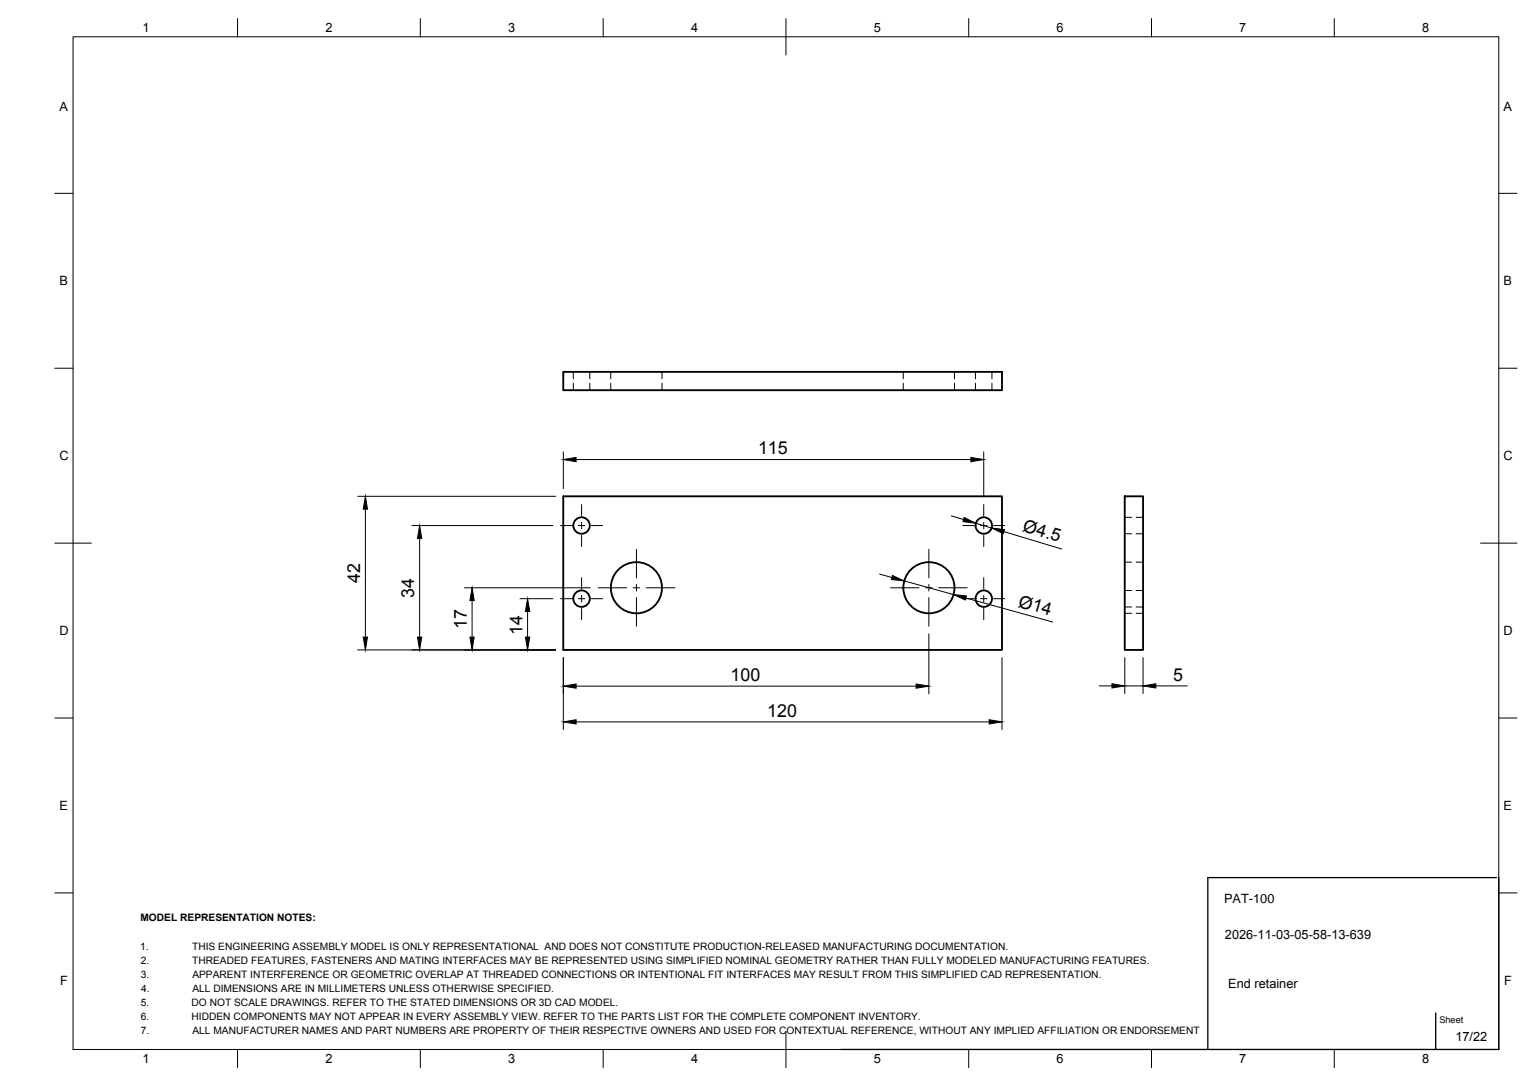
ISO-10303-21;
HEADER;
/* Generated by software containing ST-Developer
 * from STEP Tools, Inc. (www.steptools.com) 
 */

FILE_DESCRIPTION(
/* description */ (''),
/* implementation_level */ '2;1');

FILE_NAME(
/* name */ 'End retainer.step',
/* time_stamp */ '2026-10-29T16:43:51-07:00',
/* author */ (''),
/* organization */ (''),
/* preprocessor_version */ 'ST-DEVELOPER v20.2',
/* originating_system */ 'Autodesk Translation Framework v15.17.0.0',
/* authorisation */ '');

FILE_SCHEMA (('AUTOMOTIVE_DESIGN { 1 0 10303 214 3 1 1 }'));
ENDSEC;

DATA;
#10=MECHANICAL_DESIGN_GEOMETRIC_PRESENTATION_REPRESENTATION('',(#382),#10292);
#336=SHAPE_REPRESENTATION_RELATIONSHIP('SRR','None',#10434,#359);
#359=ADVANCED_BREP_SHAPE_REPRESENTATION('',(#403),#10286);
#382=STYLED_ITEM('',(#10614),#403);
#403=MANIFOLD_SOLID_BREP('Body1',#5026);
#512=FACE_BOUND('',#1329,.T.);
#513=FACE_BOUND('',#1330,.T.);
#514=FACE_BOUND('',#1331,.T.);
#515=FACE_BOUND('',#1332,.T.);
#516=FACE_BOUND('',#1333,.T.);
#517=FACE_BOUND('',#1334,.T.);
#518=FACE_BOUND('',#1337,.T.);
#519=FACE_BOUND('',#1338,.T.);
#520=FACE_BOUND('',#1339,.T.);
#521=FACE_BOUND('',#1340,.T.);
#522=FACE_BOUND('',#1341,.T.);
#523=FACE_BOUND('',#1342,.T.);
#667=PLANE('',#5702);
#668=PLANE('',#5703);
#669=PLANE('',#5704);
#670=PLANE('',#5705);
#671=PLANE('',#5706);
#672=PLANE('',#5707);
#927=FACE_OUTER_BOUND('',#1321,.T.);
#928=FACE_OUTER_BOUND('',#1322,.T.);
#929=FACE_OUTER_BOUND('',#1323,.T.);
#930=FACE_OUTER_BOUND('',#1324,.T.);
#931=FACE_OUTER_BOUND('',#1325,.T.);
#932=FACE_OUTER_BOUND('',#1326,.T.);
#933=FACE_OUTER_BOUND('',#1327,.T.);
#934=FACE_OUTER_BOUND('',#1328,.T.);
#935=FACE_OUTER_BOUND('',#1335,.T.);
#936=FACE_OUTER_BOUND('',#1336,.T.);
#937=FACE_OUTER_BOUND('',#1343,.T.);
#938=FACE_OUTER_BOUND('',#1344,.T.);
#1321=EDGE_LOOP('',(#4361,#4362,#4363,#4364));
#1322=EDGE_LOOP('',(#4365,#4366,#4367,#4368));
#1323=EDGE_LOOP('',(#4369,#4370,#4371,#4372));
#1324=EDGE_LOOP('',(#4373,#4374,#4375,#4376));
#1325=EDGE_LOOP('',(#4377,#4378,#4379,#4380));
#1326=EDGE_LOOP('',(#4381,#4382,#4383,#4384));
#1327=EDGE_LOOP('',(#4385,#4386,#4387,#4388));
#1328=EDGE_LOOP('',(#4389,#4390,#4391,#4392));
#1329=EDGE_LOOP('',(#4393));
#1330=EDGE_LOOP('',(#4394));
#1331=EDGE_LOOP('',(#4395));
#1332=EDGE_LOOP('',(#4396));
#1333=EDGE_LOOP('',(#4397));
#1334=EDGE_LOOP('',(#4398));
#1335=EDGE_LOOP('',(#4399,#4400,#4401,#4402));
#1336=EDGE_LOOP('',(#4403,#4404,#4405,#4406));
#1337=EDGE_LOOP('',(#4407));
#1338=EDGE_LOOP('',(#4408));
#1339=EDGE_LOOP('',(#4409));
#1340=EDGE_LOOP('',(#4410));
#1341=EDGE_LOOP('',(#4411));
#1342=EDGE_LOOP('',(#4412));
#1343=EDGE_LOOP('',(#4413,#4414,#4415,#4416));
#1344=EDGE_LOOP('',(#4417,#4418,#4419,#4420));
#1709=LINE('',#9879,#2101);
#1710=LINE('',#9885,#2102);
#1711=LINE('',#9891,#2103);
#1712=LINE('',#9897,#2104);
#1713=LINE('',#9903,#2105);
#1714=LINE('',#9909,#2106);
#1715=LINE('',#9914,#2107);
#1716=LINE('',#9916,#2108);
#1717=LINE('',#9918,#2109);
#1718=LINE('',#9919,#2110);
#1719=LINE('',#9922,#2111);
#1720=LINE('',#9924,#2112);
#1721=LINE('',#9925,#2113);
#1722=LINE('',#9928,#2114);
#1723=LINE('',#9930,#2115);
#1724=LINE('',#9931,#2116);
#1725=LINE('',#9933,#2117);
#1726=LINE('',#9934,#2118);
#2101=VECTOR('',#6956,0.225);
#2102=VECTOR('',#6963,0.225);
#2103=VECTOR('',#6970,0.225);
#2104=VECTOR('',#6977,0.225);
#2105=VECTOR('',#6984,0.7);
#2106=VECTOR('',#6991,0.7);
#2107=VECTOR('',#6996,1.);
#2108=VECTOR('',#6997,1.);
#2109=VECTOR('',#6998,1.);
#2110=VECTOR('',#6999,1.);
#2111=VECTOR('',#7002,1.);
#2112=VECTOR('',#7003,1.);
#2113=VECTOR('',#7004,1.);
#2114=VECTOR('',#7007,1.);
#2115=VECTOR('',#7008,1.);
#2116=VECTOR('',#7009,1.);
#2117=VECTOR('',#7012,1.);
#2118=VECTOR('',#7013,1.);
#2350=CIRCLE('',#5685,0.225);
#2351=CIRCLE('',#5686,0.225);
#2352=CIRCLE('',#5688,0.225);
#2353=CIRCLE('',#5689,0.225);
#2354=CIRCLE('',#5691,0.225);
#2355=CIRCLE('',#5692,0.225);
#2356=CIRCLE('',#5694,0.225);
#2357=CIRCLE('',#5695,0.225);
#2358=CIRCLE('',#5697,0.7);
#2359=CIRCLE('',#5698,0.7);
#2360=CIRCLE('',#5700,0.7);
#2361=CIRCLE('',#5701,0.7);
#2707=VERTEX_POINT('',#9876);
#2708=VERTEX_POINT('',#9878);
#2709=VERTEX_POINT('',#9882);
#2710=VERTEX_POINT('',#9884);
#2711=VERTEX_POINT('',#9888);
#2712=VERTEX_POINT('',#9890);
#2713=VERTEX_POINT('',#9894);
#2714=VERTEX_POINT('',#9896);
#2715=VERTEX_POINT('',#9900);
#2716=VERTEX_POINT('',#9902);
#2717=VERTEX_POINT('',#9906);
#2718=VERTEX_POINT('',#9908);
#2719=VERTEX_POINT('',#9912);
#2720=VERTEX_POINT('',#9913);
#2721=VERTEX_POINT('',#9915);
#2722=VERTEX_POINT('',#9917);
#2723=VERTEX_POINT('',#9921);
#2724=VERTEX_POINT('',#9923);
#2725=VERTEX_POINT('',#9927);
#2726=VERTEX_POINT('',#9929);
#3271=EDGE_CURVE('',#2707,#2707,#2350,.T.);
#3272=EDGE_CURVE('',#2707,#2708,#1709,.T.);
#3273=EDGE_CURVE('',#2708,#2708,#2351,.T.);
#3274=EDGE_CURVE('',#2709,#2709,#2352,.T.);
#3275=EDGE_CURVE('',#2709,#2710,#1710,.T.);
#3276=EDGE_CURVE('',#2710,#2710,#2353,.T.);
#3277=EDGE_CURVE('',#2711,#2711,#2354,.T.);
#3278=EDGE_CURVE('',#2711,#2712,#1711,.T.);
#3279=EDGE_CURVE('',#2712,#2712,#2355,.T.);
#3280=EDGE_CURVE('',#2713,#2713,#2356,.T.);
#3281=EDGE_CURVE('',#2713,#2714,#1712,.T.);
#3282=EDGE_CURVE('',#2714,#2714,#2357,.T.);
#3283=EDGE_CURVE('',#2715,#2715,#2358,.T.);
#3284=EDGE_CURVE('',#2715,#2716,#1713,.T.);
#3285=EDGE_CURVE('',#2716,#2716,#2359,.T.);
#3286=EDGE_CURVE('',#2717,#2717,#2360,.T.);
#3287=EDGE_CURVE('',#2717,#2718,#1714,.T.);
#3288=EDGE_CURVE('',#2718,#2718,#2361,.T.);
#3289=EDGE_CURVE('',#2719,#2720,#1715,.T.);
#3290=EDGE_CURVE('',#2720,#2721,#1716,.T.);
#3291=EDGE_CURVE('',#2722,#2721,#1717,.T.);
#3292=EDGE_CURVE('',#2719,#2722,#1718,.T.);
#3293=EDGE_CURVE('',#2723,#2719,#1719,.T.);
#3294=EDGE_CURVE('',#2724,#2722,#1720,.T.);
#3295=EDGE_CURVE('',#2723,#2724,#1721,.T.);
#3296=EDGE_CURVE('',#2725,#2723,#1722,.T.);
#3297=EDGE_CURVE('',#2726,#2724,#1723,.T.);
#3298=EDGE_CURVE('',#2725,#2726,#1724,.T.);
#3299=EDGE_CURVE('',#2720,#2725,#1725,.T.);
#3300=EDGE_CURVE('',#2721,#2726,#1726,.T.);
#4361=ORIENTED_EDGE('',*,*,#3271,.F.);
#4362=ORIENTED_EDGE('',*,*,#3272,.T.);
#4363=ORIENTED_EDGE('',*,*,#3273,.F.);
#4364=ORIENTED_EDGE('',*,*,#3272,.F.);
#4365=ORIENTED_EDGE('',*,*,#3274,.F.);
#4366=ORIENTED_EDGE('',*,*,#3275,.T.);
#4367=ORIENTED_EDGE('',*,*,#3276,.F.);
#4368=ORIENTED_EDGE('',*,*,#3275,.F.);
#4369=ORIENTED_EDGE('',*,*,#3277,.F.);
#4370=ORIENTED_EDGE('',*,*,#3278,.T.);
#4371=ORIENTED_EDGE('',*,*,#3279,.F.);
#4372=ORIENTED_EDGE('',*,*,#3278,.F.);
#4373=ORIENTED_EDGE('',*,*,#3280,.F.);
#4374=ORIENTED_EDGE('',*,*,#3281,.T.);
#4375=ORIENTED_EDGE('',*,*,#3282,.F.);
#4376=ORIENTED_EDGE('',*,*,#3281,.F.);
#4377=ORIENTED_EDGE('',*,*,#3283,.F.);
#4378=ORIENTED_EDGE('',*,*,#3284,.T.);
#4379=ORIENTED_EDGE('',*,*,#3285,.F.);
#4380=ORIENTED_EDGE('',*,*,#3284,.F.);
#4381=ORIENTED_EDGE('',*,*,#3286,.F.);
#4382=ORIENTED_EDGE('',*,*,#3287,.T.);
#4383=ORIENTED_EDGE('',*,*,#3288,.F.);
#4384=ORIENTED_EDGE('',*,*,#3287,.F.);
#4385=ORIENTED_EDGE('',*,*,#3289,.T.);
#4386=ORIENTED_EDGE('',*,*,#3290,.T.);
#4387=ORIENTED_EDGE('',*,*,#3291,.F.);
#4388=ORIENTED_EDGE('',*,*,#3292,.F.);
#4389=ORIENTED_EDGE('',*,*,#3293,.T.);
#4390=ORIENTED_EDGE('',*,*,#3292,.T.);
#4391=ORIENTED_EDGE('',*,*,#3294,.F.);
#4392=ORIENTED_EDGE('',*,*,#3295,.F.);
#4393=ORIENTED_EDGE('',*,*,#3288,.T.);
#4394=ORIENTED_EDGE('',*,*,#3285,.T.);
#4395=ORIENTED_EDGE('',*,*,#3282,.T.);
#4396=ORIENTED_EDGE('',*,*,#3279,.T.);
#4397=ORIENTED_EDGE('',*,*,#3276,.T.);
#4398=ORIENTED_EDGE('',*,*,#3273,.T.);
#4399=ORIENTED_EDGE('',*,*,#3296,.T.);
#4400=ORIENTED_EDGE('',*,*,#3295,.T.);
#4401=ORIENTED_EDGE('',*,*,#3297,.F.);
#4402=ORIENTED_EDGE('',*,*,#3298,.F.);
#4403=ORIENTED_EDGE('',*,*,#3299,.T.);
#4404=ORIENTED_EDGE('',*,*,#3298,.T.);
#4405=ORIENTED_EDGE('',*,*,#3300,.F.);
#4406=ORIENTED_EDGE('',*,*,#3290,.F.);
#4407=ORIENTED_EDGE('',*,*,#3286,.T.);
#4408=ORIENTED_EDGE('',*,*,#3283,.T.);
#4409=ORIENTED_EDGE('',*,*,#3280,.T.);
#4410=ORIENTED_EDGE('',*,*,#3277,.T.);
#4411=ORIENTED_EDGE('',*,*,#3274,.T.);
#4412=ORIENTED_EDGE('',*,*,#3271,.T.);
#4413=ORIENTED_EDGE('',*,*,#3300,.T.);
#4414=ORIENTED_EDGE('',*,*,#3297,.T.);
#4415=ORIENTED_EDGE('',*,*,#3294,.T.);
#4416=ORIENTED_EDGE('',*,*,#3291,.T.);
#4417=ORIENTED_EDGE('',*,*,#3299,.F.);
#4418=ORIENTED_EDGE('',*,*,#3289,.F.);
#4419=ORIENTED_EDGE('',*,*,#3293,.F.);
#4420=ORIENTED_EDGE('',*,*,#3296,.F.);
#4703=CYLINDRICAL_SURFACE('',#5684,0.225);
#4704=CYLINDRICAL_SURFACE('',#5687,0.225);
#4705=CYLINDRICAL_SURFACE('',#5690,0.225);
#4706=CYLINDRICAL_SURFACE('',#5693,0.225);
#4707=CYLINDRICAL_SURFACE('',#5696,0.7);
#4708=CYLINDRICAL_SURFACE('',#5699,0.7);
#4936=ADVANCED_FACE('',(#927),#4703,.F.);
#4937=ADVANCED_FACE('',(#928),#4704,.F.);
#4938=ADVANCED_FACE('',(#929),#4705,.F.);
#4939=ADVANCED_FACE('',(#930),#4706,.F.);
#4940=ADVANCED_FACE('',(#931),#4707,.F.);
#4941=ADVANCED_FACE('',(#932),#4708,.F.);
#4942=ADVANCED_FACE('',(#933),#667,.T.);
#4943=ADVANCED_FACE('',(#934,#512,#513,#514,#515,#516,#517),#668,.T.);
#4944=ADVANCED_FACE('',(#935),#669,.T.);
#4945=ADVANCED_FACE('',(#936,#518,#519,#520,#521,#522,#523),#670,.T.);
#4946=ADVANCED_FACE('',(#937),#671,.T.);
#4947=ADVANCED_FACE('',(#938),#672,.F.);
#5026=CLOSED_SHELL('',(#4936,#4937,#4938,#4939,#4940,#4941,#4942,#4943,
#4944,#4945,#4946,#4947));
#5683=AXIS2_PLACEMENT_3D('',#9874,#6950,#6951);
#5684=AXIS2_PLACEMENT_3D('',#9875,#6952,#6953);
#5685=AXIS2_PLACEMENT_3D('',#9877,#6954,#6955);
#5686=AXIS2_PLACEMENT_3D('',#9880,#6957,#6958);
#5687=AXIS2_PLACEMENT_3D('',#9881,#6959,#6960);
#5688=AXIS2_PLACEMENT_3D('',#9883,#6961,#6962);
#5689=AXIS2_PLACEMENT_3D('',#9886,#6964,#6965);
#5690=AXIS2_PLACEMENT_3D('',#9887,#6966,#6967);
#5691=AXIS2_PLACEMENT_3D('',#9889,#6968,#6969);
#5692=AXIS2_PLACEMENT_3D('',#9892,#6971,#6972);
#5693=AXIS2_PLACEMENT_3D('',#9893,#6973,#6974);
#5694=AXIS2_PLACEMENT_3D('',#9895,#6975,#6976);
#5695=AXIS2_PLACEMENT_3D('',#9898,#6978,#6979);
#5696=AXIS2_PLACEMENT_3D('',#9899,#6980,#6981);
#5697=AXIS2_PLACEMENT_3D('',#9901,#6982,#6983);
#5698=AXIS2_PLACEMENT_3D('',#9904,#6985,#6986);
#5699=AXIS2_PLACEMENT_3D('',#9905,#6987,#6988);
#5700=AXIS2_PLACEMENT_3D('',#9907,#6989,#6990);
#5701=AXIS2_PLACEMENT_3D('',#9910,#6992,#6993);
#5702=AXIS2_PLACEMENT_3D('',#9911,#6994,#6995);
#5703=AXIS2_PLACEMENT_3D('',#9920,#7000,#7001);
#5704=AXIS2_PLACEMENT_3D('',#9926,#7005,#7006);
#5705=AXIS2_PLACEMENT_3D('',#9932,#7010,#7011);
#5706=AXIS2_PLACEMENT_3D('',#9935,#7014,#7015);
#5707=AXIS2_PLACEMENT_3D('',#9936,#7016,#7017);
#6950=DIRECTION('axis',(0.,0.,1.));
#6951=DIRECTION('refdir',(1.,0.,0.));
#6952=DIRECTION('center_axis',(1.,0.,0.));
#6953=DIRECTION('ref_axis',(0.,0.,-1.));
#6954=DIRECTION('center_axis',(1.,0.,0.));
#6955=DIRECTION('ref_axis',(0.,0.,-1.));
#6956=DIRECTION('',(1.,0.,0.));
#6957=DIRECTION('center_axis',(-1.,0.,0.));
#6958=DIRECTION('ref_axis',(0.,0.,-1.));
#6959=DIRECTION('center_axis',(1.,0.,0.));
#6960=DIRECTION('ref_axis',(0.,0.,-1.));
#6961=DIRECTION('center_axis',(1.,0.,0.));
#6962=DIRECTION('ref_axis',(0.,0.,-1.));
#6963=DIRECTION('',(1.,0.,0.));
#6964=DIRECTION('center_axis',(-1.,0.,0.));
#6965=DIRECTION('ref_axis',(0.,0.,-1.));
#6966=DIRECTION('center_axis',(1.,0.,0.));
#6967=DIRECTION('ref_axis',(0.,0.,-1.));
#6968=DIRECTION('center_axis',(1.,0.,0.));
#6969=DIRECTION('ref_axis',(0.,0.,-1.));
#6970=DIRECTION('',(1.,0.,0.));
#6971=DIRECTION('center_axis',(-1.,0.,0.));
#6972=DIRECTION('ref_axis',(0.,0.,-1.));
#6973=DIRECTION('center_axis',(1.,0.,0.));
#6974=DIRECTION('ref_axis',(0.,0.,-1.));
#6975=DIRECTION('center_axis',(1.,0.,0.));
#6976=DIRECTION('ref_axis',(0.,0.,-1.));
#6977=DIRECTION('',(1.,0.,0.));
#6978=DIRECTION('center_axis',(-1.,0.,0.));
#6979=DIRECTION('ref_axis',(0.,0.,-1.));
#6980=DIRECTION('center_axis',(1.,0.,0.));
#6981=DIRECTION('ref_axis',(0.,0.,-1.));
#6982=DIRECTION('center_axis',(1.,0.,0.));
#6983=DIRECTION('ref_axis',(0.,0.,-1.));
#6984=DIRECTION('',(1.,0.,0.));
#6985=DIRECTION('center_axis',(-1.,0.,0.));
#6986=DIRECTION('ref_axis',(0.,0.,-1.));
#6987=DIRECTION('center_axis',(1.,0.,0.));
#6988=DIRECTION('ref_axis',(0.,0.,-1.));
#6989=DIRECTION('center_axis',(1.,0.,0.));
#6990=DIRECTION('ref_axis',(0.,0.,-1.));
#6991=DIRECTION('',(1.,0.,0.));
#6992=DIRECTION('center_axis',(-1.,0.,0.));
#6993=DIRECTION('ref_axis',(0.,0.,-1.));
#6994=DIRECTION('center_axis',(0.,1.,0.));
#6995=DIRECTION('ref_axis',(-1.,0.,0.));
#6996=DIRECTION('',(-1.,0.,0.));
#6997=DIRECTION('',(0.,0.,1.));
#6998=DIRECTION('',(-1.,0.,0.));
#6999=DIRECTION('',(0.,0.,1.));
#7000=DIRECTION('center_axis',(1.,0.,0.));
#7001=DIRECTION('ref_axis',(0.,1.,0.));
#7002=DIRECTION('',(0.,1.,0.));
#7003=DIRECTION('',(0.,1.,0.));
#7004=DIRECTION('',(0.,0.,1.));
#7005=DIRECTION('center_axis',(0.,-1.,0.));
#7006=DIRECTION('ref_axis',(1.,0.,0.));
#7007=DIRECTION('',(1.,0.,0.));
#7008=DIRECTION('',(1.,0.,0.));
#7009=DIRECTION('',(0.,0.,1.));
#7010=DIRECTION('center_axis',(-1.,0.,0.));
#7011=DIRECTION('ref_axis',(0.,-1.,0.));
#7012=DIRECTION('',(0.,-1.,0.));
#7013=DIRECTION('',(0.,-1.,0.));
#7014=DIRECTION('center_axis',(0.,0.,1.));
#7015=DIRECTION('ref_axis',(1.,0.,0.));
#7016=DIRECTION('center_axis',(0.,0.,1.));
#7017=DIRECTION('ref_axis',(1.,0.,0.));
#9874=CARTESIAN_POINT('',(0.,0.,0.));
#9875=CARTESIAN_POINT('Origin',(9.9,5.5,3.));
#9876=CARTESIAN_POINT('',(10.,5.5,3.225));
#9877=CARTESIAN_POINT('Origin',(10.,5.5,3.));
#9878=CARTESIAN_POINT('',(10.5,5.5,3.225));
#9879=CARTESIAN_POINT('',(9.9,5.5,3.225));
#9880=CARTESIAN_POINT('Origin',(10.5,5.5,3.));
#9881=CARTESIAN_POINT('Origin',(9.9,-5.5,5.));
#9882=CARTESIAN_POINT('',(10.,-5.5,5.225));
#9883=CARTESIAN_POINT('Origin',(10.,-5.5,5.));
#9884=CARTESIAN_POINT('',(10.5,-5.5,5.225));
#9885=CARTESIAN_POINT('',(9.9,-5.5,5.225));
#9886=CARTESIAN_POINT('Origin',(10.5,-5.5,5.));
#9887=CARTESIAN_POINT('Origin',(9.9,-5.5,3.));
#9888=CARTESIAN_POINT('',(10.,-5.5,3.225));
#9889=CARTESIAN_POINT('Origin',(10.,-5.5,3.));
#9890=CARTESIAN_POINT('',(10.5,-5.5,3.225));
#9891=CARTESIAN_POINT('',(9.9,-5.5,3.225));
#9892=CARTESIAN_POINT('Origin',(10.5,-5.5,3.));
#9893=CARTESIAN_POINT('Origin',(9.9,5.5,5.));
#9894=CARTESIAN_POINT('',(10.,5.5,5.225));
#9895=CARTESIAN_POINT('Origin',(10.,5.5,5.));
#9896=CARTESIAN_POINT('',(10.5,5.5,5.225));
#9897=CARTESIAN_POINT('',(9.9,5.5,5.225));
#9898=CARTESIAN_POINT('Origin',(10.5,5.5,5.));
#9899=CARTESIAN_POINT('Origin',(9.9,-4.,3.3));
#9900=CARTESIAN_POINT('',(10.,-4.,4.));
#9901=CARTESIAN_POINT('Origin',(10.,-4.,3.3));
#9902=CARTESIAN_POINT('',(10.5,-4.,4.));
#9903=CARTESIAN_POINT('',(9.9,-4.,4.));
#9904=CARTESIAN_POINT('Origin',(10.5,-4.,3.3));
#9905=CARTESIAN_POINT('Origin',(9.9,4.,3.3));
#9906=CARTESIAN_POINT('',(10.,4.,4.));
#9907=CARTESIAN_POINT('Origin',(10.,4.,3.3));
#9908=CARTESIAN_POINT('',(10.5,4.,4.));
#9909=CARTESIAN_POINT('',(9.9,4.,4.));
#9910=CARTESIAN_POINT('Origin',(10.5,4.,3.3));
#9911=CARTESIAN_POINT('Origin',(10.5,6.,1.6));
#9912=CARTESIAN_POINT('',(10.5,6.,1.6));
#9913=CARTESIAN_POINT('',(10.,6.,1.6));
#9914=CARTESIAN_POINT('',(10.5,6.,1.6));
#9915=CARTESIAN_POINT('',(10.,6.,5.8));
#9916=CARTESIAN_POINT('',(10.,6.,1.6));
#9917=CARTESIAN_POINT('',(10.5,6.,5.8));
#9918=CARTESIAN_POINT('',(10.5,6.,5.8));
#9919=CARTESIAN_POINT('',(10.5,6.,1.6));
#9920=CARTESIAN_POINT('Origin',(10.5,-6.,1.6));
#9921=CARTESIAN_POINT('',(10.5,-6.,1.6));
#9922=CARTESIAN_POINT('',(10.5,-6.,1.6));
#9923=CARTESIAN_POINT('',(10.5,-6.,5.8));
#9924=CARTESIAN_POINT('',(10.5,-6.,5.8));
#9925=CARTESIAN_POINT('',(10.5,-6.,1.6));
#9926=CARTESIAN_POINT('Origin',(10.,-6.,1.6));
#9927=CARTESIAN_POINT('',(10.,-6.,1.6));
#9928=CARTESIAN_POINT('',(10.,-6.,1.6));
#9929=CARTESIAN_POINT('',(10.,-6.,5.8));
#9930=CARTESIAN_POINT('',(10.,-6.,5.8));
#9931=CARTESIAN_POINT('',(10.,-6.,1.6));
#9932=CARTESIAN_POINT('Origin',(10.,6.,1.6));
#9933=CARTESIAN_POINT('',(10.,6.,1.6));
#9934=CARTESIAN_POINT('',(10.,6.,5.8));
#9935=CARTESIAN_POINT('Origin',(10.25,0.,5.8));
#9936=CARTESIAN_POINT('Origin',(10.25,0.,1.6));
#10258=UNCERTAINTY_MEASURE_WITH_UNIT(LENGTH_MEASURE(0.001),#10293,
'DISTANCE_ACCURACY_VALUE',
'Maximum model space distance between geometric entities at asserted c
onnectivities');
#10264=UNCERTAINTY_MEASURE_WITH_UNIT(LENGTH_MEASURE(0.001),#10293,
'DISTANCE_ACCURACY_VALUE',
'Maximum model space distance between geometric entities at asserted c
onnectivities');
#10286=(
GEOMETRIC_REPRESENTATION_CONTEXT(3)
GLOBAL_UNCERTAINTY_ASSIGNED_CONTEXT((#10258))
GLOBAL_UNIT_ASSIGNED_CONTEXT((#10293,#10295,#10296))
REPRESENTATION_CONTEXT('','3D')
);
#10292=(
GEOMETRIC_REPRESENTATION_CONTEXT(3)
GLOBAL_UNCERTAINTY_ASSIGNED_CONTEXT((#10264))
GLOBAL_UNIT_ASSIGNED_CONTEXT((#10293,#10295,#10296))
REPRESENTATION_CONTEXT('','3D')
);
#10293=(
LENGTH_UNIT()
NAMED_UNIT(*)
SI_UNIT(.CENTI.,.METRE.)
);
#10295=(
NAMED_UNIT(*)
PLANE_ANGLE_UNIT()
SI_UNIT($,.RADIAN.)
);
#10296=(
NAMED_UNIT(*)
SI_UNIT($,.STERADIAN.)
SOLID_ANGLE_UNIT()
);
#10318=SHAPE_DEFINITION_REPRESENTATION(#10347,#10434);
#10347=PRODUCT_DEFINITION_SHAPE('',$,#10462);
#10434=SHAPE_REPRESENTATION('',(#5683),#10286);
#10440=PRODUCT_DEFINITION_CONTEXT('part definition',#10523,'design');
#10462=PRODUCT_DEFINITION('End retainer','End retainer',#10489,
#10440);
#10489=PRODUCT_DEFINITION_FORMATION('',$,#10546);
#10523=APPLICATION_CONTEXT(
'Core Data for Automotive Mechanical Design Process');
#10524=PRODUCT_CONTEXT('part definition',#10523,'mechanical');
#10546=PRODUCT('End retainer','End retainer','End retainer',
(#10524));
#10608=COLOUR_RGB('Light Blue',0.38,0.62,0.78);
#10609=FILL_AREA_STYLE_COLOUR('',#10608);
#10610=FILL_AREA_STYLE('',(#10609));
#10611=SURFACE_STYLE_FILL_AREA(#10610);
#10612=SURFACE_SIDE_STYLE('',(#10611));
#10613=SURFACE_STYLE_USAGE(.BOTH.,#10612);
#10614=PRESENTATION_STYLE_ASSIGNMENT((#10613));
ENDSEC;
END-ISO-10303-21;
